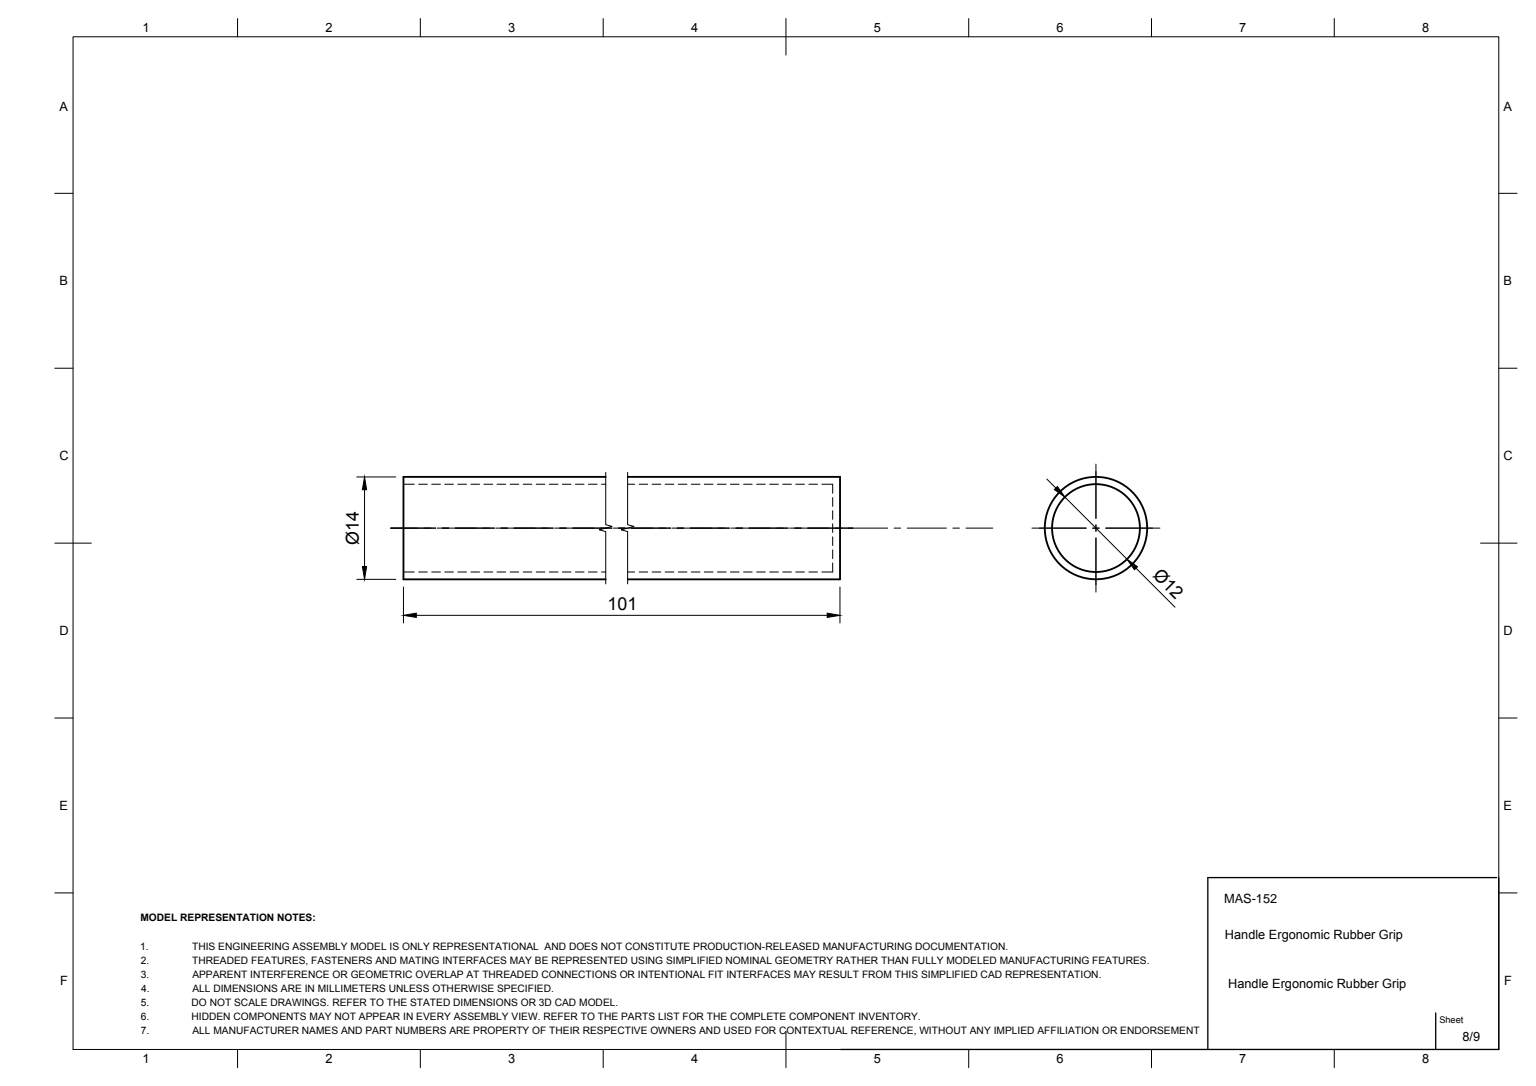
ISO-10303-21;
HEADER;
/* Generated by software containing ST-Developer
 * from STEP Tools, Inc. (www.steptools.com) 
 */

FILE_DESCRIPTION(
/* description */ ('STEP AP214'),
/* implementation_level */ '2;1');

FILE_NAME(
/* name */ 'Handle Ergonomic Rubber Grip.step',
/* time_stamp */ '2026-11-04T19:18:53-08:00',
/* author */ (''),
/* organization */ (''),
/* preprocessor_version */ 'ST-DEVELOPER v20.2',
/* originating_system */ 'Autodesk Translation Framework v15.17.0.0',
/* authorisation */ '');

FILE_SCHEMA (('AUTOMOTIVE_DESIGN { 1 0 10303 214 3 1 1 }'));
ENDSEC;

DATA;
#10=MECHANICAL_DESIGN_GEOMETRIC_PRESENTATION_REPRESENTATION('',(#83),#5942);
#69=SHAPE_REPRESENTATION_RELATIONSHIP('SRR','None',#5980,#76);
#76=ADVANCED_BREP_SHAPE_REPRESENTATION('',(#90),#5940);
#83=STYLED_ITEM('',(#6020),#90);
#90=MANIFOLD_SOLID_BREP('Body1',#930);
#97=FACE_BOUND('',#242,.T.);
#129=PLANE('',#1085);
#130=PLANE('',#1086);
#131=PLANE('',#1087);
#180=FACE_OUTER_BOUND('',#239,.T.);
#181=FACE_OUTER_BOUND('',#240,.T.);
#182=FACE_OUTER_BOUND('',#241,.T.);
#183=FACE_OUTER_BOUND('',#243,.T.);
#184=FACE_OUTER_BOUND('',#244,.T.);
#239=EDGE_LOOP('',(#808,#809,#810,#811));
#240=EDGE_LOOP('',(#812,#813,#814,#815));
#241=EDGE_LOOP('',(#816));
#242=EDGE_LOOP('',(#817));
#243=EDGE_LOOP('',(#818));
#244=EDGE_LOOP('',(#819));
#313=LINE('',#5858,#391);
#314=LINE('',#5864,#392);
#391=VECTOR('',#1310,6.);
#392=VECTOR('',#1317,7.);
#438=CIRCLE('',#1080,6.);
#439=CIRCLE('',#1081,6.);
#440=CIRCLE('',#1083,7.);
#441=CIRCLE('',#1084,7.);
#502=VERTEX_POINT('',#5855);
#503=VERTEX_POINT('',#5857);
#504=VERTEX_POINT('',#5861);
#505=VERTEX_POINT('',#5863);
#607=EDGE_CURVE('',#502,#502,#438,.T.);
#608=EDGE_CURVE('',#502,#503,#313,.T.);
#609=EDGE_CURVE('',#503,#503,#439,.T.);
#610=EDGE_CURVE('',#504,#504,#440,.T.);
#611=EDGE_CURVE('',#504,#505,#314,.T.);
#612=EDGE_CURVE('',#505,#505,#441,.T.);
#808=ORIENTED_EDGE('',*,*,#607,.F.);
#809=ORIENTED_EDGE('',*,*,#608,.T.);
#810=ORIENTED_EDGE('',*,*,#609,.T.);
#811=ORIENTED_EDGE('',*,*,#608,.F.);
#812=ORIENTED_EDGE('',*,*,#610,.F.);
#813=ORIENTED_EDGE('',*,*,#611,.T.);
#814=ORIENTED_EDGE('',*,*,#612,.T.);
#815=ORIENTED_EDGE('',*,*,#611,.F.);
#816=ORIENTED_EDGE('',*,*,#612,.F.);
#817=ORIENTED_EDGE('',*,*,#607,.T.);
#818=ORIENTED_EDGE('',*,*,#610,.T.);
#819=ORIENTED_EDGE('',*,*,#609,.F.);
#868=CYLINDRICAL_SURFACE('',#1079,6.);
#869=CYLINDRICAL_SURFACE('',#1082,7.);
#911=ADVANCED_FACE('',(#180),#868,.F.);
#912=ADVANCED_FACE('',(#181),#869,.T.);
#913=ADVANCED_FACE('',(#182,#97),#129,.T.);
#914=ADVANCED_FACE('',(#183),#130,.T.);
#915=ADVANCED_FACE('',(#184),#131,.F.);
#930=CLOSED_SHELL('',(#911,#912,#913,#914,#915));
#1078=AXIS2_PLACEMENT_3D('',#5853,#1304,#1305);
#1079=AXIS2_PLACEMENT_3D('',#5854,#1306,#1307);
#1080=AXIS2_PLACEMENT_3D('',#5856,#1308,#1309);
#1081=AXIS2_PLACEMENT_3D('',#5859,#1311,#1312);
#1082=AXIS2_PLACEMENT_3D('',#5860,#1313,#1314);
#1083=AXIS2_PLACEMENT_3D('',#5862,#1315,#1316);
#1084=AXIS2_PLACEMENT_3D('',#5865,#1318,#1319);
#1085=AXIS2_PLACEMENT_3D('',#5866,#1320,#1321);
#1086=AXIS2_PLACEMENT_3D('',#5867,#1322,#1323);
#1087=AXIS2_PLACEMENT_3D('',#5868,#1324,#1325);
#1304=DIRECTION('axis',(0.,0.,1.));
#1305=DIRECTION('refdir',(1.,0.,0.));
#1306=DIRECTION('center_axis',(1.38777878078145E-16,-1.,0.));
#1307=DIRECTION('ref_axis',(1.,1.38777878078145E-16,0.));
#1308=DIRECTION('center_axis',(1.56125112837913E-16,-1.,0.));
#1309=DIRECTION('ref_axis',(1.,1.56125112837913E-16,0.));
#1310=DIRECTION('',(1.38777878078145E-16,-1.,0.));
#1311=DIRECTION('center_axis',(1.56125112837913E-16,-1.,0.));
#1312=DIRECTION('ref_axis',(1.,1.56125112837913E-16,0.));
#1313=DIRECTION('center_axis',(1.38777878078145E-16,-1.,0.));
#1314=DIRECTION('ref_axis',(1.,1.38777878078145E-16,0.));
#1315=DIRECTION('center_axis',(1.56125112837913E-16,-1.,0.));
#1316=DIRECTION('ref_axis',(1.,1.56125112837913E-16,0.));
#1317=DIRECTION('',(-1.38777878078145E-16,1.,0.));
#1318=DIRECTION('center_axis',(1.38777878078145E-16,-1.,0.));
#1319=DIRECTION('ref_axis',(1.,1.38777878078145E-16,0.));
#1320=DIRECTION('center_axis',(-1.56125112837913E-16,1.,0.));
#1321=DIRECTION('ref_axis',(-1.,-1.56125112837913E-16,0.));
#1322=DIRECTION('center_axis',(1.56125112837913E-16,-1.,0.));
#1323=DIRECTION('ref_axis',(1.,1.56125112837913E-16,0.));
#1324=DIRECTION('center_axis',(1.56125112837913E-16,-1.,0.));
#1325=DIRECTION('ref_axis',(1.,1.56125112837913E-16,0.));
#5853=CARTESIAN_POINT('',(0.,0.,0.));
#5854=CARTESIAN_POINT('Origin',(11.4999999999999,-32.3205080756888,0.));
#5855=CARTESIAN_POINT('',(5.49999999999991,-32.3205080756888,-7.34788079488412E-16));
#5856=CARTESIAN_POINT('Origin',(11.4999999999999,-32.3205080756888,0.));
#5857=CARTESIAN_POINT('',(5.49999999999992,-132.320508075689,-7.34788079488412E-16));
#5858=CARTESIAN_POINT('',(5.49999999999991,-32.3205080756888,-7.34788079488412E-16));
#5859=CARTESIAN_POINT('Origin',(11.4999999999999,-132.320508075689,0.));
#5860=CARTESIAN_POINT('Origin',(11.4999999999999,-32.3205080756888,0.));
#5861=CARTESIAN_POINT('',(4.49999999999992,-133.320508075689,-8.57252759403147E-16));
#5862=CARTESIAN_POINT('Origin',(11.4999999999999,-133.320508075689,0.));
#5863=CARTESIAN_POINT('',(4.49999999999991,-32.3205080756888,-8.57252759403147E-16));
#5864=CARTESIAN_POINT('',(4.49999999999991,-32.3205080756888,-8.57252759403147E-16));
#5865=CARTESIAN_POINT('Origin',(11.4999999999999,-32.3205080756888,0.));
#5866=CARTESIAN_POINT('Origin',(11.4999999999999,-32.3205080756888,0.));
#5867=CARTESIAN_POINT('Origin',(11.4999999999999,-133.320508075689,0.));
#5868=CARTESIAN_POINT('Origin',(11.4999999999999,-132.320508075689,0.));
#5931=UNCERTAINTY_MEASURE_WITH_UNIT(LENGTH_MEASURE(0.01),#5943,
'DISTANCE_ACCURACY_VALUE',
'Maximum model space distance between geometric entities at asserted c
onnectivities');
#5933=UNCERTAINTY_MEASURE_WITH_UNIT(LENGTH_MEASURE(0.01),#5943,
'DISTANCE_ACCURACY_VALUE',
'Maximum model space distance between geometric entities at asserted c
onnectivities');
#5940=(
GEOMETRIC_REPRESENTATION_CONTEXT(3)
GLOBAL_UNCERTAINTY_ASSIGNED_CONTEXT((#5931))
GLOBAL_UNIT_ASSIGNED_CONTEXT((#5943,#5945,#5946))
REPRESENTATION_CONTEXT('','3D')
);
#5942=(
GEOMETRIC_REPRESENTATION_CONTEXT(3)
GLOBAL_UNCERTAINTY_ASSIGNED_CONTEXT((#5933))
GLOBAL_UNIT_ASSIGNED_CONTEXT((#5943,#5945,#5946))
REPRESENTATION_CONTEXT('','3D')
);
#5943=(
LENGTH_UNIT()
NAMED_UNIT(*)
SI_UNIT(.MILLI.,.METRE.)
);
#5945=(
NAMED_UNIT(*)
PLANE_ANGLE_UNIT()
SI_UNIT($,.RADIAN.)
);
#5946=(
NAMED_UNIT(*)
SI_UNIT($,.STERADIAN.)
SOLID_ANGLE_UNIT()
);
#5953=SHAPE_DEFINITION_REPRESENTATION(#5961,#5980);
#5961=PRODUCT_DEFINITION_SHAPE('',$,#5989);
#5980=SHAPE_REPRESENTATION('',(#1078),#5940);
#5982=PRODUCT_DEFINITION_CONTEXT('part definition',#6008,'design');
#5989=PRODUCT_DEFINITION('Handle Ergonomic Rubber Grip',
'Handle Ergonomic Rubber Grip',#5997,#5982);
#5997=PRODUCT_DEFINITION_FORMATION('',$,#6016);
#6008=APPLICATION_CONTEXT(
'Core Data for Automotive Mechanical Design Process');
#6009=PRODUCT_CONTEXT('part definition',#6008,'mechanical');
#6016=PRODUCT('Handle Ergonomic Rubber Grip',
'Handle Ergonomic Rubber Grip',$,(#6009));
#6020=PRESENTATION_STYLE_ASSIGNMENT((#6026));
#6026=SURFACE_STYLE_USAGE(.BOTH.,#6032);
#6032=SURFACE_SIDE_STYLE('',(#6038));
#6038=SURFACE_STYLE_FILL_AREA(#6044);
#6044=FILL_AREA_STYLE('Opaque(31,36,43)',(#6050));
#6050=FILL_AREA_STYLE_COLOUR('Opaque(31,36,43)',#6056);
#6056=COLOUR_RGB('Opaque(31,36,43)',0.12156862745098,0.141176470588235,
0.168627450980392);
ENDSEC;
END-ISO-10303-21;
